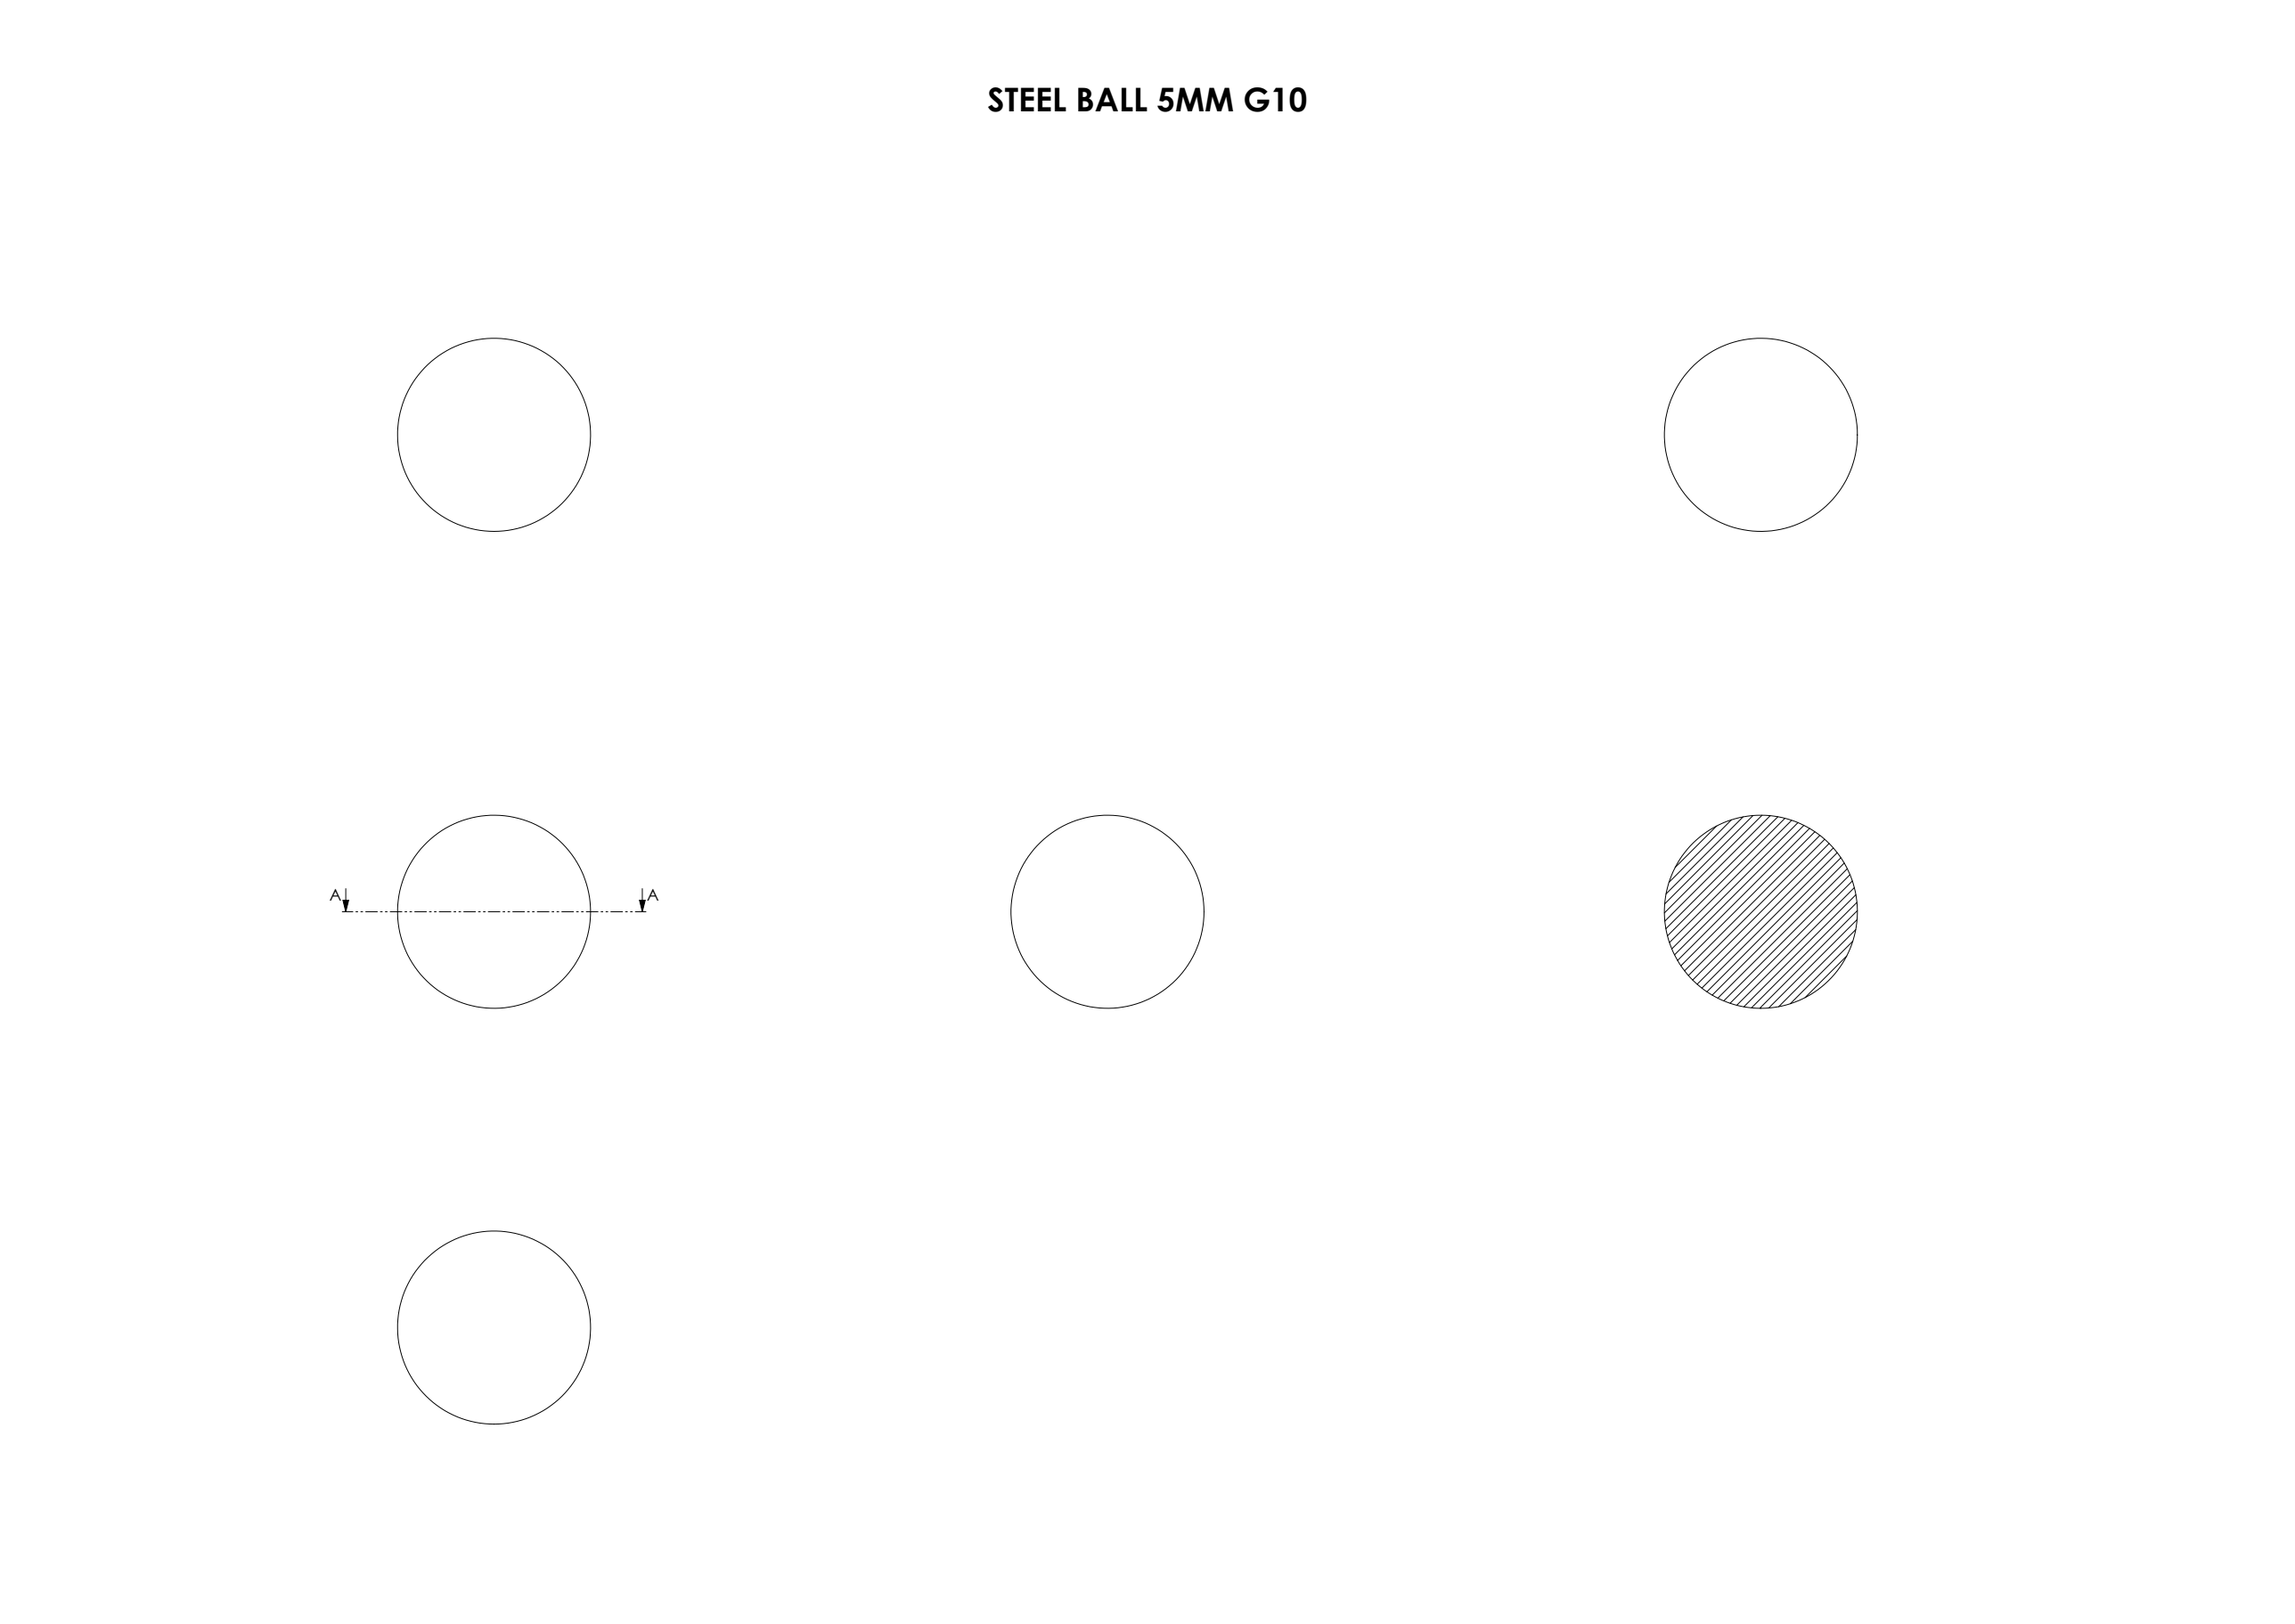
ISO-10303-21;
HEADER;
/* Generated by software containing ST-Developer
 * from STEP Tools, Inc. (www.steptools.com) 
 */

FILE_DESCRIPTION(
/* description */ (''),
/* implementation_level */ '2;1');

FILE_NAME(
/* name */ '03_Steel_Ball_5mm_G10.step',
/* time_stamp */ '2026-10-11T08:53:36-07:00',
/* author */ (''),
/* organization */ (''),
/* preprocessor_version */ 'ST-DEVELOPER v20.2',
/* originating_system */ 'Autodesk Translation Framework v15.15.0.0',
/* authorisation */ '');

FILE_SCHEMA (('AUTOMOTIVE_DESIGN { 1 0 10303 214 3 1 1 }'));
ENDSEC;

DATA;
#10=MECHANICAL_DESIGN_GEOMETRIC_PRESENTATION_REPRESENTATION('',(#74),#3338);
#63=SPHERICAL_SURFACE('',#1793,2.5);
#66=SHAPE_REPRESENTATION_RELATIONSHIP('SRR','None',#3369,#70);
#70=ADVANCED_BREP_SHAPE_REPRESENTATION('',(#78),#3336);
#74=STYLED_ITEM('',(#3443),#78);
#78=MANIFOLD_SOLID_BREP('Body1',#1576);
#277=FACE_OUTER_BOUND('',#399,.T.);
#399=EDGE_LOOP('',(#1428,#1429));
#679=CIRCLE('',#1794,2.5);
#808=VERTEX_POINT('',#3294);
#809=VERTEX_POINT('',#3295);
#1016=EDGE_CURVE('',#808,#809,#679,.T.);
#1428=ORIENTED_EDGE('',*,*,#1016,.T.);
#1429=ORIENTED_EDGE('',*,*,#1016,.F.);
#1568=ADVANCED_FACE('',(#277),#63,.T.);
#1576=CLOSED_SHELL('',(#1568));
#1792=AXIS2_PLACEMENT_3D('',#3292,#2250,#2251);
#1793=AXIS2_PLACEMENT_3D('',#3293,#2252,#2253);
#1794=AXIS2_PLACEMENT_3D('',#3296,#2254,#2255);
#2250=DIRECTION('axis',(0.,0.,1.));
#2251=DIRECTION('refdir',(1.,0.,0.));
#2252=DIRECTION('center_axis',(6.12323399573677E-17,0.,1.));
#2253=DIRECTION('ref_axis',(1.,0.,0.));
#2254=DIRECTION('center_axis',(1.22464679914735E-16,-1.,0.));
#2255=DIRECTION('ref_axis',(-1.,-1.22464679914735E-16,0.));
#3292=CARTESIAN_POINT('',(0.,0.,0.));
#3293=CARTESIAN_POINT('Origin',(0.,0.,0.));
#3294=CARTESIAN_POINT('',(-1.53080849893419E-16,-1.87469972832732E-32,2.5));
#3295=CARTESIAN_POINT('',(-1.53080849893419E-16,-1.87469972832732E-32,-2.5));
#3296=CARTESIAN_POINT('Origin',(0.,0.,0.));
#3330=UNCERTAINTY_MEASURE_WITH_UNIT(LENGTH_MEASURE(0.01),#3339,
'DISTANCE_ACCURACY_VALUE',
'Maximum model space distance between geometric entities at asserted c
onnectivities');
#3332=UNCERTAINTY_MEASURE_WITH_UNIT(LENGTH_MEASURE(0.01),#3339,
'DISTANCE_ACCURACY_VALUE',
'Maximum model space distance between geometric entities at asserted c
onnectivities');
#3336=(
GEOMETRIC_REPRESENTATION_CONTEXT(3)
GLOBAL_UNCERTAINTY_ASSIGNED_CONTEXT((#3330))
GLOBAL_UNIT_ASSIGNED_CONTEXT((#3339,#3341,#3342))
REPRESENTATION_CONTEXT('','3D')
);
#3338=(
GEOMETRIC_REPRESENTATION_CONTEXT(3)
GLOBAL_UNCERTAINTY_ASSIGNED_CONTEXT((#3332))
GLOBAL_UNIT_ASSIGNED_CONTEXT((#3339,#3341,#3342))
REPRESENTATION_CONTEXT('','3D')
);
#3339=(
LENGTH_UNIT()
NAMED_UNIT(*)
SI_UNIT(.MILLI.,.METRE.)
);
#3341=(
NAMED_UNIT(*)
PLANE_ANGLE_UNIT()
SI_UNIT($,.RADIAN.)
);
#3342=(
NAMED_UNIT(*)
SI_UNIT($,.STERADIAN.)
SOLID_ANGLE_UNIT()
);
#3346=SHAPE_DEFINITION_REPRESENTATION(#3351,#3369);
#3351=PRODUCT_DEFINITION_SHAPE('',$,#3375);
#3369=SHAPE_REPRESENTATION('',(#1792),#3336);
#3371=PRODUCT_DEFINITION_CONTEXT('part definition',#3388,'design');
#3375=PRODUCT_DEFINITION('2026-10-11-08-53-16-659',
'03_Steel_Ball_5mm_G10',#3380,#3371);
#3380=PRODUCT_DEFINITION_FORMATION('',$,#3393);
#3388=APPLICATION_CONTEXT(
'Core Data for Automotive Mechanical Design Process');
#3389=PRODUCT_CONTEXT('part definition',#3388,'mechanical');
#3393=PRODUCT('2026-10-11-08-53-16-659','03_Steel_Ball_5mm_G10',$,(#3389));
#3437=COLOUR_RGB('Light Blue',0.38,0.62,0.78);
#3438=FILL_AREA_STYLE_COLOUR('',#3437);
#3439=FILL_AREA_STYLE('',(#3438));
#3440=SURFACE_STYLE_FILL_AREA(#3439);
#3441=SURFACE_SIDE_STYLE('',(#3440));
#3442=SURFACE_STYLE_USAGE(.BOTH.,#3441);
#3443=PRESENTATION_STYLE_ASSIGNMENT((#3442));
ENDSEC;
END-ISO-10303-21;
